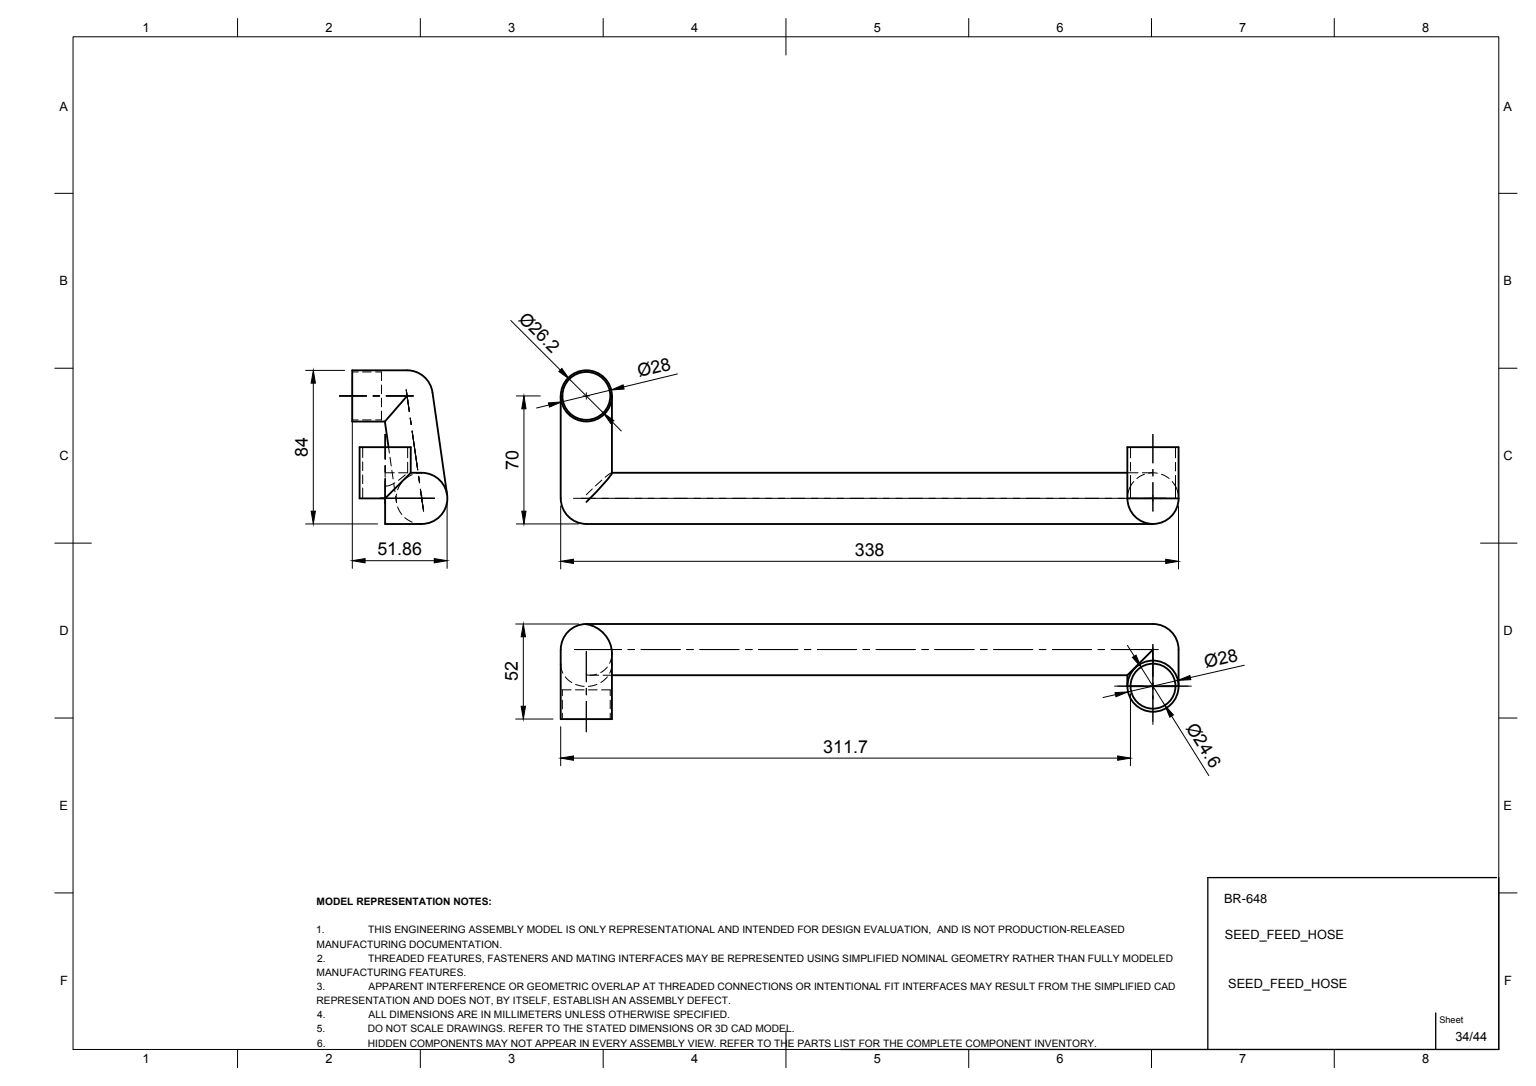
ISO-10303-21;
HEADER;
FILE_DESCRIPTION((''),'2;1');
FILE_NAME('SEED_FEED_HOSE.step','2026-10-01T22:05:39-07:00',(''),(''),'','','');
FILE_SCHEMA (('AUTOMOTIVE_DESIGN { 1 0 10303 214 3 1 1 }'));
ENDSEC;
DATA;
#10=MECHANICAL_DESIGN_GEOMETRIC_PRESENTATION_REPRESENTATION('',(#632),#24628);
#353=ELLIPSE('',#15108,1.97989898732233,1.4) ;
#354=ELLIPSE('',#15114,1.97989898732233,1.4) ;
#355=ELLIPSE('',#15116,1.97989898732233,1.4) ;
#356=ELLIPSE('',#15134,1.97989898732233,1.4) ;
#357=ELLIPSE('',#15135,1.97989898732233,1.4) ;
#358=ELLIPSE('',#15137,1.85319037744393,1.4) ;
#482=SPHERICAL_SURFACE('',#15121,1.4) ;
#483=SPHERICAL_SURFACE('',#15123,1.4) ;
#484=SPHERICAL_SURFACE('',#15129,1.4) ;
#548=SHAPE_REPRESENTATION_RELATIONSHIP('SRR','None',#24821,#590) ;
#590=ADVANCED_BREP_SHAPE_REPRESENTATION('',(#671),#24611) ;
#632=STYLED_ITEM('',(#25033),#671) ;
#671=MANIFOLD_SOLID_BREP('SEED_FEED_HOSE',#13174) ;
#902=FACE_BOUND('',#4577,.T.) ;
#903=FACE_BOUND('',#4590,.T.) ;
#984=B_SPLINE_CURVE_WITH_KNOTS('',3,(#23620,#23621,#23622,#23623,#23624,
#23625,#23626,#23627,#23628,#23629,#23630,#23631,#23632,#23633,#23634,#23635,
#23636,#23637,#23638,#23639,#23640,#23641,#23642,#23643,#23644,#23645,#23646,
#23647,#23648,#23649),.UNSPECIFIED.,.F.,.F.,(4,2,2,2,2,2,2,2,2,2,2,2,2,
2,4),(-4.08940558183937,-3.82598745493601,-3.56256932803264,-3.29915120112928,
-3.03573307422591,-2.5402179325728,-2.29246036174624,-2.04470279091969,
-1.79694522009313,-1.54918764926658,-1.05367250761347,-0.7902543807101,
-0.526836253806733,-0.263418126903367,0.),.UNSPECIFIED.) ;
#1668=LINE('',#23601,#2504) ;
#1669=LINE('',#23605,#2505) ;
#1670=LINE('',#23610,#2506) ;
#1671=LINE('',#23614,#2507) ;
#1672=LINE('',#23616,#2508) ;
#1673=LINE('',#23618,#2509) ;
#1674=LINE('',#23654,#2510) ;
#1675=LINE('',#23686,#2511) ;
#1676=LINE('',#23690,#2512) ;
#1677=LINE('',#23694,#2513) ;
#1678=LINE('',#23699,#2514) ;
#2504=VECTOR('',#18961,1.) ;
#2505=VECTOR('',#18964,1.) ;
#2506=VECTOR('',#18971,1.4) ;
#2507=VECTOR('',#18976,1.) ;
#2508=VECTOR('',#18977,1.) ;
#2509=VECTOR('',#18978,1.23) ;
#2510=VECTOR('',#18987,1.4) ;
#2511=VECTOR('',#19028,1.4) ;
#2512=VECTOR('',#19035,1.4) ;
#2513=VECTOR('',#19040,1.31) ;
#2514=VECTOR('',#19047,1.4) ;
#2905=CYLINDRICAL_SURFACE('',#15106,1.4) ;
#2906=CYLINDRICAL_SURFACE('',#15109,1.23) ;
#2907=CYLINDRICAL_SURFACE('',#15112,1.4) ;
#2908=CYLINDRICAL_SURFACE('',#15117,1.4) ;
#2909=CYLINDRICAL_SURFACE('',#15133,1.4) ;
#2910=CYLINDRICAL_SURFACE('',#15136,1.4) ;
#2911=CYLINDRICAL_SURFACE('',#15138,1.31) ;
#2912=CYLINDRICAL_SURFACE('',#15140,1.4) ;
#3590=FACE_OUTER_BOUND('',#4573,.T.) ;
#3591=FACE_OUTER_BOUND('',#4574,.T.) ;
#3592=FACE_OUTER_BOUND('',#4575,.T.) ;
#3593=FACE_OUTER_BOUND('',#4576,.T.) ;
#3594=FACE_OUTER_BOUND('',#4578,.T.) ;
#3595=FACE_OUTER_BOUND('',#4579,.T.) ;
#3596=FACE_OUTER_BOUND('',#4580,.T.) ;
#3597=FACE_OUTER_BOUND('',#4581,.T.) ;
#3598=FACE_OUTER_BOUND('',#4582,.T.) ;
#3599=FACE_OUTER_BOUND('',#4583,.T.) ;
#3600=FACE_OUTER_BOUND('',#4584,.T.) ;
#3601=FACE_OUTER_BOUND('',#4585,.T.) ;
#3602=FACE_OUTER_BOUND('',#4586,.T.) ;
#3603=FACE_OUTER_BOUND('',#4587,.T.) ;
#3604=FACE_OUTER_BOUND('',#4588,.T.) ;
#3605=FACE_OUTER_BOUND('',#4589,.T.) ;
#4573=EDGE_LOOP('',(#11423,#11424,#11425,#11426)) ;
#4574=EDGE_LOOP('',(#11427,#11428,#11429,#11430,#11431)) ;
#4575=EDGE_LOOP('',(#11432,#11433,#11434,#11435,#11436,#11437,#11438)) ;
#4576=EDGE_LOOP('',(#11439)) ;
#4577=EDGE_LOOP('',(#11440)) ;
#4578=EDGE_LOOP('',(#11441,#11442,#11443,#11444,#11445,#11446,#11447)) ;
#4579=EDGE_LOOP('',(#11448,#11449)) ;
#4580=EDGE_LOOP('',(#11450)) ;
#4581=EDGE_LOOP('',(#11451,#11452)) ;
#4582=EDGE_LOOP('',(#11453,#11454,#11455,#11456,#11457,#11458)) ;
#4583=EDGE_LOOP('',(#11459,#11460)) ;
#4584=EDGE_LOOP('',(#11461,#11462,#11463,#11464,#11465,#11466)) ;
#4585=EDGE_LOOP('',(#11467,#11468,#11469,#11470,#11471,#11472,#11473,#11474,
#11475)) ;
#4586=EDGE_LOOP('',(#11476,#11477,#11478,#11479,#11480,#11481,#11482,#11483)) ;
#4587=EDGE_LOOP('',(#11484,#11485,#11486,#11487)) ;
#4588=EDGE_LOOP('',(#11488,#11489,#11490,#11491,#11492)) ;
#4589=EDGE_LOOP('',(#11493)) ;
#4590=EDGE_LOOP('',(#11494)) ;
#5443=CIRCLE('',#15104,1.4) ;
#5444=CIRCLE('',#15105,1.23) ;
#5445=CIRCLE('',#15107,1.4) ;
#5446=CIRCLE('',#15110,1.23) ;
#5447=CIRCLE('',#15113,1.4) ;
#5448=CIRCLE('',#15115,1.4) ;
#5449=CIRCLE('',#15118,1.4) ;
#5450=CIRCLE('',#15120,1.31) ;
#5451=CIRCLE('',#15122,1.4) ;
#5452=CIRCLE('',#15124,1.4) ;
#5453=CIRCLE('',#15125,1.4) ;
#5454=CIRCLE('',#15126,1.4) ;
#5455=CIRCLE('',#15127,1.4) ;
#5456=CIRCLE('',#15128,1.4) ;
#5457=CIRCLE('',#15130,1.4) ;
#5458=CIRCLE('',#15131,1.4) ;
#5459=CIRCLE('',#15139,1.31) ;
#5460=CIRCLE('',#15141,1.4) ;
#6545=VERTEX_POINT('',#23599) ;
#6546=VERTEX_POINT('',#23600) ;
#6547=VERTEX_POINT('',#23602) ;
#6548=VERTEX_POINT('',#23604) ;
#6549=VERTEX_POINT('',#23608) ;
#6550=VERTEX_POINT('',#23613) ;
#6551=VERTEX_POINT('',#23615) ;
#6552=VERTEX_POINT('',#23617) ;
#6553=VERTEX_POINT('',#23653) ;
#6554=VERTEX_POINT('',#23655) ;
#6555=VERTEX_POINT('',#23657) ;
#6556=VERTEX_POINT('',#23663) ;
#6557=VERTEX_POINT('',#23668) ;
#6558=VERTEX_POINT('',#23669) ;
#6559=VERTEX_POINT('',#23671) ;
#6560=VERTEX_POINT('',#23673) ;
#6561=VERTEX_POINT('',#23675) ;
#6562=VERTEX_POINT('',#23679) ;
#6563=VERTEX_POINT('',#23680) ;
#6564=VERTEX_POINT('',#23685) ;
#6565=VERTEX_POINT('',#23693) ;
#6566=VERTEX_POINT('',#23697) ;
#8201=EDGE_CURVE('',#6545,#6546,#1668,.T.) ;
#8202=EDGE_CURVE('',#6545,#6547,#5443,.T.) ;
#8203=EDGE_CURVE('',#6548,#6547,#1669,.T.) ;
#8204=EDGE_CURVE('',#6548,#6546,#5444,.T.) ;
#8205=EDGE_CURVE('',#6549,#6549,#5445,.T.) ;
#8206=EDGE_CURVE('',#6549,#6547,#1670,.T.) ;
#8207=EDGE_CURVE('',#6547,#6545,#353,.T.) ;
#8208=EDGE_CURVE('',#6546,#6550,#1671,.T.) ;
#8209=EDGE_CURVE('',#6551,#6548,#1672,.T.) ;
#8210=EDGE_CURVE('',#6551,#6552,#1673,.T.) ;
#8211=EDGE_CURVE('',#6552,#6552,#5446,.T.) ;
#8212=EDGE_CURVE('',#6550,#6551,#984,.T.) ;
#8213=EDGE_CURVE('',#6547,#6545,#5447,.T.) ;
#8214=EDGE_CURVE('',#6547,#6553,#1674,.T.) ;
#8215=EDGE_CURVE('',#6554,#6553,#354,.T.) ;
#8216=EDGE_CURVE('',#6555,#6554,#5448,.T.) ;
#8217=EDGE_CURVE('',#6553,#6555,#355,.T.) ;
#8218=EDGE_CURVE('',#6550,#6551,#5449,.T.) ;
#8219=EDGE_CURVE('',#6556,#6556,#5450,.T.) ;
#8220=EDGE_CURVE('',#6554,#6555,#5451,.T.) ;
#8221=EDGE_CURVE('',#6557,#6558,#5452,.T.) ;
#8222=EDGE_CURVE('',#6558,#6559,#5453,.T.) ;
#8223=EDGE_CURVE('',#6558,#6560,#5454,.T.) ;
#8224=EDGE_CURVE('',#6560,#6561,#5455,.T.) ;
#8225=EDGE_CURVE('',#6561,#6557,#5456,.T.) ;
#8226=EDGE_CURVE('',#6562,#6563,#5457,.T.) ;
#8227=EDGE_CURVE('',#6563,#6562,#5458,.T.) ;
#8228=EDGE_CURVE('',#6553,#6564,#1675,.T.) ;
#8229=EDGE_CURVE('',#6560,#6564,#356,.T.) ;
#8230=EDGE_CURVE('',#6564,#6557,#357,.T.) ;
#8231=EDGE_CURVE('',#6561,#6563,#1676,.T.) ;
#8232=EDGE_CURVE('',#6563,#6562,#358,.T.) ;
#8233=EDGE_CURVE('',#6556,#6565,#1677,.T.) ;
#8234=EDGE_CURVE('',#6565,#6565,#5459,.T.) ;
#8235=EDGE_CURVE('',#6566,#6566,#5460,.T.) ;
#8236=EDGE_CURVE('',#6566,#6563,#1678,.T.) ;
#11423=ORIENTED_EDGE('',*,*,#8201,.F.) ;
#11424=ORIENTED_EDGE('',*,*,#8202,.T.) ;
#11425=ORIENTED_EDGE('',*,*,#8203,.F.) ;
#11426=ORIENTED_EDGE('',*,*,#8204,.T.) ;
#11427=ORIENTED_EDGE('',*,*,#8205,.F.) ;
#11428=ORIENTED_EDGE('',*,*,#8206,.T.) ;
#11429=ORIENTED_EDGE('',*,*,#8202,.F.) ;
#11430=ORIENTED_EDGE('',*,*,#8207,.F.) ;
#11431=ORIENTED_EDGE('',*,*,#8206,.F.) ;
#11432=ORIENTED_EDGE('',*,*,#8208,.F.) ;
#11433=ORIENTED_EDGE('',*,*,#8204,.F.) ;
#11434=ORIENTED_EDGE('',*,*,#8209,.F.) ;
#11435=ORIENTED_EDGE('',*,*,#8210,.T.) ;
#11436=ORIENTED_EDGE('',*,*,#8211,.F.) ;
#11437=ORIENTED_EDGE('',*,*,#8210,.F.) ;
#11438=ORIENTED_EDGE('',*,*,#8212,.F.) ;
#11439=ORIENTED_EDGE('',*,*,#8205,.T.) ;
#11440=ORIENTED_EDGE('',*,*,#8211,.T.) ;
#11441=ORIENTED_EDGE('',*,*,#8207,.T.) ;
#11442=ORIENTED_EDGE('',*,*,#8213,.F.) ;
#11443=ORIENTED_EDGE('',*,*,#8214,.T.) ;
#11444=ORIENTED_EDGE('',*,*,#8215,.F.) ;
#11445=ORIENTED_EDGE('',*,*,#8216,.F.) ;
#11446=ORIENTED_EDGE('',*,*,#8217,.F.) ;
#11447=ORIENTED_EDGE('',*,*,#8214,.F.) ;
#11448=ORIENTED_EDGE('',*,*,#8212,.T.) ;
#11449=ORIENTED_EDGE('',*,*,#8218,.F.) ;
#11450=ORIENTED_EDGE('',*,*,#8219,.T.) ;
#11451=ORIENTED_EDGE('',*,*,#8216,.T.) ;
#11452=ORIENTED_EDGE('',*,*,#8220,.T.) ;
#11453=ORIENTED_EDGE('',*,*,#8221,.T.) ;
#11454=ORIENTED_EDGE('',*,*,#8222,.T.) ;
#11455=ORIENTED_EDGE('',*,*,#8222,.F.) ;
#11456=ORIENTED_EDGE('',*,*,#8223,.T.) ;
#11457=ORIENTED_EDGE('',*,*,#8224,.T.) ;
#11458=ORIENTED_EDGE('',*,*,#8225,.T.) ;
#11459=ORIENTED_EDGE('',*,*,#8226,.T.) ;
#11460=ORIENTED_EDGE('',*,*,#8227,.T.) ;
#11461=ORIENTED_EDGE('',*,*,#8208,.T.) ;
#11462=ORIENTED_EDGE('',*,*,#8218,.T.) ;
#11463=ORIENTED_EDGE('',*,*,#8209,.T.) ;
#11464=ORIENTED_EDGE('',*,*,#8203,.T.) ;
#11465=ORIENTED_EDGE('',*,*,#8213,.T.) ;
#11466=ORIENTED_EDGE('',*,*,#8201,.T.) ;
#11467=ORIENTED_EDGE('',*,*,#8215,.T.) ;
#11468=ORIENTED_EDGE('',*,*,#8228,.T.) ;
#11469=ORIENTED_EDGE('',*,*,#8229,.F.) ;
#11470=ORIENTED_EDGE('',*,*,#8223,.F.) ;
#11471=ORIENTED_EDGE('',*,*,#8221,.F.) ;
#11472=ORIENTED_EDGE('',*,*,#8230,.F.) ;
#11473=ORIENTED_EDGE('',*,*,#8228,.F.) ;
#11474=ORIENTED_EDGE('',*,*,#8217,.T.) ;
#11475=ORIENTED_EDGE('',*,*,#8220,.F.) ;
#11476=ORIENTED_EDGE('',*,*,#8229,.T.) ;
#11477=ORIENTED_EDGE('',*,*,#8230,.T.) ;
#11478=ORIENTED_EDGE('',*,*,#8225,.F.) ;
#11479=ORIENTED_EDGE('',*,*,#8231,.T.) ;
#11480=ORIENTED_EDGE('',*,*,#8226,.F.) ;
#11481=ORIENTED_EDGE('',*,*,#8232,.F.) ;
#11482=ORIENTED_EDGE('',*,*,#8231,.F.) ;
#11483=ORIENTED_EDGE('',*,*,#8224,.F.) ;
#11484=ORIENTED_EDGE('',*,*,#8219,.F.) ;
#11485=ORIENTED_EDGE('',*,*,#8233,.T.) ;
#11486=ORIENTED_EDGE('',*,*,#8234,.F.) ;
#11487=ORIENTED_EDGE('',*,*,#8233,.F.) ;
#11488=ORIENTED_EDGE('',*,*,#8235,.F.) ;
#11489=ORIENTED_EDGE('',*,*,#8236,.T.) ;
#11490=ORIENTED_EDGE('',*,*,#8232,.T.) ;
#11491=ORIENTED_EDGE('',*,*,#8227,.F.) ;
#11492=ORIENTED_EDGE('',*,*,#8236,.F.) ;
#11493=ORIENTED_EDGE('',*,*,#8235,.T.) ;
#11494=ORIENTED_EDGE('',*,*,#8234,.T.) ;
#12270=PLANE('',#15103) ;
#12271=PLANE('',#15111) ;
#12272=PLANE('',#15119) ;
#12273=PLANE('',#15132) ;
#12274=PLANE('',#15142) ;
#12985=ADVANCED_FACE('',(#3590),#12270,.T.) ;
#12986=ADVANCED_FACE('',(#3591),#2905,.T.) ;
#12987=ADVANCED_FACE('',(#3592),#2906,.F.) ;
#12988=ADVANCED_FACE('',(#3593,#902),#12271,.T.) ;
#12989=ADVANCED_FACE('',(#3594),#2907,.T.) ;
#12990=ADVANCED_FACE('',(#3595),#2908,.T.) ;
#12991=ADVANCED_FACE('',(#3596),#12272,.T.) ;
#12992=ADVANCED_FACE('',(#3597),#482,.T.) ;
#12993=ADVANCED_FACE('',(#3598),#483,.T.) ;
#12994=ADVANCED_FACE('',(#3599),#484,.T.) ;
#12995=ADVANCED_FACE('',(#3600),#12273,.T.) ;
#12996=ADVANCED_FACE('',(#3601),#2909,.T.) ;
#12997=ADVANCED_FACE('',(#3602),#2910,.T.) ;
#12998=ADVANCED_FACE('',(#3603),#2911,.F.) ;
#12999=ADVANCED_FACE('',(#3604),#2912,.T.) ;
#13000=ADVANCED_FACE('',(#3605,#903),#12274,.T.) ;
#13174=CLOSED_SHELL('',(#12985,#12986,#12987,#12988,#12989,#12990,#12991,
#12992,#12993,#12994,#12995,#12996,#12997,#12998,#12999,#13000)) ;
#15102=AXIS2_PLACEMENT_3D('',#23597,#18957,#18958) ;
#15103=AXIS2_PLACEMENT_3D('',#23598,#18959,#18960) ;
#15104=AXIS2_PLACEMENT_3D('',#23603,#18962,#18963) ;
#15105=AXIS2_PLACEMENT_3D('',#23606,#18965,#18966) ;
#15106=AXIS2_PLACEMENT_3D('',#23607,#18967,#18968) ;
#15107=AXIS2_PLACEMENT_3D('',#23609,#18969,#18970) ;
#15108=AXIS2_PLACEMENT_3D('',#23611,#18972,#18973) ;
#15109=AXIS2_PLACEMENT_3D('',#23612,#18974,#18975) ;
#15110=AXIS2_PLACEMENT_3D('',#23619,#18979,#18980) ;
#15111=AXIS2_PLACEMENT_3D('',#23650,#18981,#18982) ;
#15112=AXIS2_PLACEMENT_3D('',#23651,#18983,#18984) ;
#15113=AXIS2_PLACEMENT_3D('',#23652,#18985,#18986) ;
#15114=AXIS2_PLACEMENT_3D('',#23656,#18988,#18989) ;
#15115=AXIS2_PLACEMENT_3D('',#23658,#18990,#18991) ;
#15116=AXIS2_PLACEMENT_3D('',#23659,#18992,#18993) ;
#15117=AXIS2_PLACEMENT_3D('',#23660,#18994,#18995) ;
#15118=AXIS2_PLACEMENT_3D('',#23661,#18996,#18997) ;
#15119=AXIS2_PLACEMENT_3D('',#23662,#18998,#18999) ;
#15120=AXIS2_PLACEMENT_3D('',#23664,#19000,#19001) ;
#15121=AXIS2_PLACEMENT_3D('',#23665,#19002,#19003) ;
#15122=AXIS2_PLACEMENT_3D('',#23666,#19004,#19005) ;
#15123=AXIS2_PLACEMENT_3D('',#23667,#19006,#19007) ;
#15124=AXIS2_PLACEMENT_3D('',#23670,#19008,#19009) ;
#15125=AXIS2_PLACEMENT_3D('',#23672,#19010,#19011) ;
#15126=AXIS2_PLACEMENT_3D('',#23674,#19012,#19013) ;
#15127=AXIS2_PLACEMENT_3D('',#23676,#19014,#19015) ;
#15128=AXIS2_PLACEMENT_3D('',#23677,#19016,#19017) ;
#15129=AXIS2_PLACEMENT_3D('',#23678,#19018,#19019) ;
#15130=AXIS2_PLACEMENT_3D('',#23681,#19020,#19021) ;
#15131=AXIS2_PLACEMENT_3D('',#23682,#19022,#19023) ;
#15132=AXIS2_PLACEMENT_3D('',#23683,#19024,#19025) ;
#15133=AXIS2_PLACEMENT_3D('',#23684,#19026,#19027) ;
#15134=AXIS2_PLACEMENT_3D('',#23687,#19029,#19030) ;
#15135=AXIS2_PLACEMENT_3D('',#23688,#19031,#19032) ;
#15136=AXIS2_PLACEMENT_3D('',#23689,#19033,#19034) ;
#15137=AXIS2_PLACEMENT_3D('',#23691,#19036,#19037) ;
#15138=AXIS2_PLACEMENT_3D('',#23692,#19038,#19039) ;
#15139=AXIS2_PLACEMENT_3D('',#23695,#19041,#19042) ;
#15140=AXIS2_PLACEMENT_3D('',#23696,#19043,#19044) ;
#15141=AXIS2_PLACEMENT_3D('',#23698,#19045,#19046) ;
#15142=AXIS2_PLACEMENT_3D('',#23700,#19048,#19049) ;
#18957=DIRECTION('axis',(0.,0.,1.)) ;
#18958=DIRECTION('refdir',(1.,0.,0.)) ;
#18959=DIRECTION('center_axis',(0.,-1.,0.)) ;
#18960=DIRECTION('ref_axis',(-1.,0.,0.)) ;
#18961=DIRECTION('',(-1.,0.,0.)) ;
#18962=DIRECTION('center_axis',(0.,-1.,0.)) ;
#18963=DIRECTION('ref_axis',(1.,0.,0.)) ;
#18964=DIRECTION('',(-1.,0.,0.)) ;
#18965=DIRECTION('center_axis',(0.,1.,0.)) ;
#18966=DIRECTION('ref_axis',(1.,0.,0.)) ;
#18967=DIRECTION('center_axis',(0.,1.,0.)) ;
#18968=DIRECTION('ref_axis',(1.,0.,0.)) ;
#18969=DIRECTION('center_axis',(0.,1.,0.)) ;
#18970=DIRECTION('ref_axis',(1.,0.,0.)) ;
#18971=DIRECTION('',(0.,-1.,0.)) ;
#18972=DIRECTION('center_axis',(0.,-0.707106781186548,-0.707106781186548)) ;
#18973=DIRECTION('ref_axis',(0.,0.707106781186547,-0.707106781186547)) ;
#18974=DIRECTION('center_axis',(0.,1.,0.)) ;
#18975=DIRECTION('ref_axis',(1.,0.,0.)) ;
#18976=DIRECTION('',(0.,1.,0.)) ;
#18977=DIRECTION('',(0.,-1.,0.)) ;
#18978=DIRECTION('',(0.,1.,0.)) ;
#18979=DIRECTION('center_axis',(0.,-1.,0.)) ;
#18980=DIRECTION('ref_axis',(1.,0.,0.)) ;
#18981=DIRECTION('center_axis',(0.,1.,0.)) ;
#18982=DIRECTION('ref_axis',(1.,0.,0.)) ;
#18983=DIRECTION('center_axis',(0.,0.,1.)) ;
#18984=DIRECTION('ref_axis',(1.,0.,0.)) ;
#18985=DIRECTION('center_axis',(0.,0.,1.)) ;
#18986=DIRECTION('ref_axis',(1.,0.,0.)) ;
#18987=DIRECTION('',(0.,0.,-1.)) ;
#18988=DIRECTION('center_axis',(-0.707106781186548,0.,-0.707106781186547)) ;
#18989=DIRECTION('ref_axis',(0.707106781186547,0.,-0.707106781186548)) ;
#18990=DIRECTION('center_axis',(0.,0.,-1.)) ;
#18991=DIRECTION('ref_axis',(1.,0.,0.)) ;
#18992=DIRECTION('center_axis',(-0.707106781186548,0.,-0.707106781186547)) ;
#18993=DIRECTION('ref_axis',(0.707106781186547,0.,-0.707106781186548)) ;
#18994=DIRECTION('center_axis',(0.,0.,1.)) ;
#18995=DIRECTION('ref_axis',(1.,0.,0.)) ;
#18996=DIRECTION('center_axis',(0.,0.,1.)) ;
#18997=DIRECTION('ref_axis',(1.,0.,0.)) ;
#18998=DIRECTION('center_axis',(0.,0.,1.)) ;
#18999=DIRECTION('ref_axis',(-1.,0.,0.)) ;
#19000=DIRECTION('center_axis',(0.,0.,1.)) ;
#19001=DIRECTION('ref_axis',(1.,0.,0.)) ;
#19002=DIRECTION('center_axis',(0.577350269189627,0.577350269189626,0.577350269189625)) ;
#19003=DIRECTION('ref_axis',(0.707106781186548,0.,-0.707106781186548)) ;
#19004=DIRECTION('center_axis',(1.,0.,0.)) ;
#19005=DIRECTION('ref_axis',(0.,0.,-1.)) ;
#19006=DIRECTION('center_axis',(0.577350269189625,0.577350269189626,0.577350269189627)) ;
#19007=DIRECTION('ref_axis',(-0.707106781186548,0.,0.707106781186547)) ;
#19008=DIRECTION('center_axis',(-1.,0.,0.)) ;
#19009=DIRECTION('ref_axis',(0.,0.,-1.)) ;
#19010=DIRECTION('center_axis',(-0.408248290463863,0.816496580927726,-0.408248290463863)) ;
#19011=DIRECTION('ref_axis',(0.707106781186548,0.,-0.707106781186547)) ;
#19012=DIRECTION('center_axis',(-1.,0.,0.)) ;
#19013=DIRECTION('ref_axis',(0.,0.,-1.)) ;
#19014=DIRECTION('center_axis',(0.,-0.989949493661167,-0.141421356237309)) ;
#19015=DIRECTION('ref_axis',(1.,0.,0.)) ;
#19016=DIRECTION('center_axis',(0.,-0.989949493661167,-0.141421356237309)) ;
#19017=DIRECTION('ref_axis',(1.,0.,0.)) ;
#19018=DIRECTION('center_axis',(0.,0.,1.)) ;
#19019=DIRECTION('ref_axis',(1.,0.,0.)) ;
#19020=DIRECTION('center_axis',(0.,0.989949493661167,0.141421356237309)) ;
#19021=DIRECTION('ref_axis',(1.,0.,0.)) ;
#19022=DIRECTION('center_axis',(0.,0.,-1.)) ;
#19023=DIRECTION('ref_axis',(1.,0.,0.)) ;
#19024=DIRECTION('center_axis',(0.,0.,1.)) ;
#19025=DIRECTION('ref_axis',(1.,0.,0.)) ;
#19026=DIRECTION('center_axis',(1.,0.,0.)) ;
#19027=DIRECTION('ref_axis',(0.,0.,-1.)) ;
#19028=DIRECTION('',(-1.,0.,0.)) ;
#19029=DIRECTION('center_axis',(-0.707106781186548,0.7,0.1)) ;
#19030=DIRECTION('ref_axis',(-0.707106781186547,-0.7,-0.1)) ;
#19031=DIRECTION('center_axis',(-0.707106781186548,0.7,0.1)) ;
#19032=DIRECTION('ref_axis',(-0.707106781186547,-0.7,-0.1)) ;
#19033=DIRECTION('center_axis',(0.,-0.989949493661167,-0.141421356237309)) ;
#19034=DIRECTION('ref_axis',(1.,0.,0.)) ;
#19035=DIRECTION('',(0.,0.989949493661167,0.141421356237309)) ;
#19036=DIRECTION('center_axis',(0.,0.655201741360129,0.755453954995706)) ;
#19037=DIRECTION('ref_axis',(0.,-0.755453954995706,0.655201741360129)) ;
#19038=DIRECTION('center_axis',(0.,0.,1.)) ;
#19039=DIRECTION('ref_axis',(1.,0.,0.)) ;
#19040=DIRECTION('',(0.,0.,1.)) ;
#19041=DIRECTION('center_axis',(0.,0.,-1.)) ;
#19042=DIRECTION('ref_axis',(1.,0.,0.)) ;
#19043=DIRECTION('center_axis',(0.,0.,1.)) ;
#19044=DIRECTION('ref_axis',(1.,0.,0.)) ;
#19045=DIRECTION('center_axis',(0.,0.,1.)) ;
#19046=DIRECTION('ref_axis',(1.,0.,0.)) ;
#19047=DIRECTION('',(0.,0.,-1.)) ;
#19048=DIRECTION('center_axis',(0.,0.,1.)) ;
#19049=DIRECTION('ref_axis',(1.,0.,0.)) ;
#23597=CARTESIAN_POINT('',(0.,0.,0.)) ;
#23598=CARTESIAN_POINT('Origin',(8.,-7.4,-8.)) ;
#23599=CARTESIAN_POINT('',(9.4,-7.4,-8.)) ;
#23600=CARTESIAN_POINT('',(9.23,-7.4,-8.)) ;
#23601=CARTESIAN_POINT('',(8.,-7.4,-8.)) ;
#23602=CARTESIAN_POINT('',(6.6,-7.4,-8.)) ;
#23603=CARTESIAN_POINT('Origin',(8.,-7.4,-8.)) ;
#23604=CARTESIAN_POINT('',(6.77,-7.4,-8.)) ;
#23605=CARTESIAN_POINT('',(8.,-7.4,-8.)) ;
#23606=CARTESIAN_POINT('Origin',(8.,-7.4,-8.)) ;
#23607=CARTESIAN_POINT('Origin',(8.,-6.,-8.)) ;
#23608=CARTESIAN_POINT('',(6.6,-4.6,-8.)) ;
#23609=CARTESIAN_POINT('Origin',(8.,-4.6,-8.)) ;
#23610=CARTESIAN_POINT('',(6.6,-6.,-8.)) ;
#23611=CARTESIAN_POINT('Origin',(8.,-7.4,-8.)) ;
#23612=CARTESIAN_POINT('Origin',(8.,-6.,-8.)) ;
#23613=CARTESIAN_POINT('',(9.23,-6.73134463286384,-8.)) ;
#23614=CARTESIAN_POINT('',(9.23,-6.,-8.)) ;
#23615=CARTESIAN_POINT('',(6.77,-6.73134463286384,-8.)) ;
#23616=CARTESIAN_POINT('',(6.77,-6.,-8.)) ;
#23617=CARTESIAN_POINT('',(6.77,-4.6,-8.)) ;
#23618=CARTESIAN_POINT('',(6.77,-6.,-8.)) ;
#23619=CARTESIAN_POINT('Origin',(8.,-4.6,-8.)) ;
#23620=CARTESIAN_POINT('Ctrl Pts',(9.23,-6.73134463286384,-8.)) ;
#23621=CARTESIAN_POINT('Ctrl Pts',(9.23,-6.73134463286384,-8.08780604230112)) ;
#23622=CARTESIAN_POINT('Ctrl Pts',(9.22072799863506,-6.71377567825997,-8.17157966039377)) ;
#23623=CARTESIAN_POINT('Ctrl Pts',(9.18717385924031,-6.65723564339427,-8.33201605328968)) ;
#23624=CARTESIAN_POINT('Ctrl Pts',(9.16282342807417,-6.61855579361812,-8.40876702722022)) ;
#23625=CARTESIAN_POINT('Ctrl Pts',(9.10036397056989,-6.53281362355673,-8.55538171579166)) ;
#23626=CARTESIAN_POINT('Ctrl Pts',(9.06220933130718,-6.48575698731823,-8.62513175063278)) ;
#23627=CARTESIAN_POINT('Ctrl Pts',(8.97399636293542,-6.39229962882938,-8.75525456150379)) ;
#23628=CARTESIAN_POINT('Ctrl Pts',(8.92390015166212,-6.3458722876066,-8.81558253005679)) ;
#23629=CARTESIAN_POINT('Ctrl Pts',(8.76786334513407,-6.22216790150124,-8.97161933658483)) ;
#23630=CARTESIAN_POINT('Ctrl Pts',(8.63606117977349,-6.14254167736889,-9.06545127512159)) ;
#23631=CARTESIAN_POINT('Ctrl Pts',(8.41018345337793,-6.05903266002601,-9.16248210994164)) ;
#23632=CARTESIAN_POINT('Ctrl Pts',(8.33024026117397,-6.03696421286031,-9.18778520433019)) ;
#23633=CARTESIAN_POINT('Ctrl Pts',(8.16644432291491,-6.00744067465883,-9.22155172186516)) ;
#23634=CARTESIAN_POINT('Ctrl Pts',(8.08258585694218,-6.,-9.23)) ;
#23635=CARTESIAN_POINT('Ctrl Pts',(7.91741414305782,-6.,-9.23)) ;
#23636=CARTESIAN_POINT('Ctrl Pts',(7.83355567708509,-6.00744067465883,-9.22155172186516)) ;
#23637=CARTESIAN_POINT('Ctrl Pts',(7.66975973882603,-6.0369642128603,-9.18778520433019)) ;
#23638=CARTESIAN_POINT('Ctrl Pts',(7.58981654662208,-6.05903266002601,-9.16248210994164)) ;
#23639=CARTESIAN_POINT('Ctrl Pts',(7.36393882022652,-6.14254167736889,-9.06545127512159)) ;
#23640=CARTESIAN_POINT('Ctrl Pts',(7.23213665486593,-6.22216790150124,-8.97161933658483)) ;
#23641=CARTESIAN_POINT('Ctrl Pts',(7.07609984833788,-6.3458722876066,-8.81558253005679)) ;
#23642=CARTESIAN_POINT('Ctrl Pts',(7.02600363706458,-6.39229962882937,-8.75525456150379)) ;
#23643=CARTESIAN_POINT('Ctrl Pts',(6.93779066869282,-6.48575698731822,-8.62513175063279)) ;
#23644=CARTESIAN_POINT('Ctrl Pts',(6.89963602943012,-6.53281362355673,-8.55538171579166)) ;
#23645=CARTESIAN_POINT('Ctrl Pts',(6.83717657192583,-6.61855579361812,-8.40876702722023)) ;
#23646=CARTESIAN_POINT('Ctrl Pts',(6.81282614075969,-6.65723564339427,-8.33201605328968)) ;
#23647=CARTESIAN_POINT('Ctrl Pts',(6.77927200136494,-6.71377567825997,-8.17157966039377)) ;
#23648=CARTESIAN_POINT('Ctrl Pts',(6.77,-6.73134463286384,-8.08780604230112)) ;
#23649=CARTESIAN_POINT('Ctrl Pts',(6.77,-6.73134463286384,-8.)) ;
#23650=CARTESIAN_POINT('Origin',(8.,-4.6,-8.)) ;
#23651=CARTESIAN_POINT('Origin',(8.,-7.4,-9.)) ;
#23652=CARTESIAN_POINT('Origin',(8.,-7.4,-8.)) ;
#23653=CARTESIAN_POINT('',(6.6,-7.4,-8.6)) ;
#23654=CARTESIAN_POINT('',(6.6,-7.4,-9.)) ;
#23655=CARTESIAN_POINT('',(8.,-8.8,-10.)) ;
#23656=CARTESIAN_POINT('Origin',(8.,-7.4,-10.)) ;
#23657=CARTESIAN_POINT('',(8.,-6.,-10.)) ;
#23658=CARTESIAN_POINT('Origin',(8.,-7.4,-10.)) ;
#23659=CARTESIAN_POINT('Origin',(8.,-7.4,-10.)) ;
#23660=CARTESIAN_POINT('Origin',(8.,-7.4,-9.)) ;
#23661=CARTESIAN_POINT('Origin',(8.,-7.4,-8.)) ;
#23662=CARTESIAN_POINT('Origin',(-23.,-1.8,-7.8)) ;
#23663=CARTESIAN_POINT('',(-24.31,-1.8,-7.8)) ;
#23664=CARTESIAN_POINT('Origin',(-23.,-1.8,-7.8)) ;
#23665=CARTESIAN_POINT('Origin',(8.,-7.4,-10.)) ;
#23666=CARTESIAN_POINT('Origin',(8.,-7.4,-10.)) ;
#23667=CARTESIAN_POINT('Origin',(-23.,-7.4,-10.)) ;
#23668=CARTESIAN_POINT('',(-23.,-7.20201010126786,-11.3859292911256)) ;
#23669=CARTESIAN_POINT('',(-23.,-8.02609903369994,-11.2521980673999)) ;
#23670=CARTESIAN_POINT('Origin',(-23.,-7.4,-10.)) ;
#23671=CARTESIAN_POINT('',(-23.8082903768655,-8.20829037686548,-10.8082903768655)) ;
#23672=CARTESIAN_POINT('Origin',(-23.,-7.4,-10.)) ;
#23673=CARTESIAN_POINT('',(-23.,-7.59798989873238,-8.61407070887439)) ;
#23674=CARTESIAN_POINT('Origin',(-23.,-7.4,-10.)) ;
#23675=CARTESIAN_POINT('',(-24.4,-7.40000000000007,-10.)) ;
#23676=CARTESIAN_POINT('Origin',(-23.,-7.4,-10.)) ;
#23677=CARTESIAN_POINT('Origin',(-23.,-7.4,-10.)) ;
#23678=CARTESIAN_POINT('Origin',(-23.,-1.8,-9.2)) ;
#23679=CARTESIAN_POINT('',(-21.6,-1.8,-9.2)) ;
#23680=CARTESIAN_POINT('',(-24.4,-1.8,-9.2)) ;
#23681=CARTESIAN_POINT('Origin',(-23.,-1.8,-9.2)) ;
#23682=CARTESIAN_POINT('Origin',(-23.,-1.8,-9.2)) ;
#23683=CARTESIAN_POINT('Origin',(8.,-7.4,-8.)) ;
#23684=CARTESIAN_POINT('Origin',(-7.5,-7.4,-10.)) ;
#23685=CARTESIAN_POINT('',(-22.8020101012678,-7.4,-8.6)) ;
#23686=CARTESIAN_POINT('',(-7.5,-7.4,-8.6)) ;
#23687=CARTESIAN_POINT('Origin',(-23.,-7.4,-10.)) ;
#23688=CARTESIAN_POINT('Origin',(-23.,-7.4,-10.)) ;
#23689=CARTESIAN_POINT('Origin',(-23.,-4.6,-9.6)) ;
#23690=CARTESIAN_POINT('',(-24.4,-4.6,-9.6)) ;
#23691=CARTESIAN_POINT('Origin',(-23.,-1.8,-9.2)) ;
#23692=CARTESIAN_POINT('Origin',(-23.,-1.8,-7.)) ;
#23693=CARTESIAN_POINT('',(-24.31,-1.8,-6.2)) ;
#23694=CARTESIAN_POINT('',(-24.31,-1.8,-7.)) ;
#23695=CARTESIAN_POINT('Origin',(-23.,-1.8,-6.2)) ;
#23696=CARTESIAN_POINT('Origin',(-23.,-1.8,-7.)) ;
#23697=CARTESIAN_POINT('',(-24.4,-1.8,-6.2)) ;
#23698=CARTESIAN_POINT('Origin',(-23.,-1.8,-6.2)) ;
#23699=CARTESIAN_POINT('',(-24.4,-1.8,-7.)) ;
#23700=CARTESIAN_POINT('Origin',(-23.,-1.8,-6.2)) ;
#24563=UNCERTAINTY_MEASURE_WITH_UNIT(LENGTH_MEASURE(0.001),#24629,
'DISTANCE_ACCURACY_VALUE',
'Maximum model space distance between geometric entities at asserted c
onnectivities') ;
#24580=UNCERTAINTY_MEASURE_WITH_UNIT(LENGTH_MEASURE(0.001),#24629,
'DISTANCE_ACCURACY_VALUE',
'Maximum model space distance between geometric entities at asserted c
onnectivities') ;
#24611=(
GEOMETRIC_REPRESENTATION_CONTEXT(3)
GLOBAL_UNCERTAINTY_ASSIGNED_CONTEXT((#24563))
GLOBAL_UNIT_ASSIGNED_CONTEXT((#24629,#24631,#24632))
REPRESENTATION_CONTEXT('','3D')
) ;
#24628=(
GEOMETRIC_REPRESENTATION_CONTEXT(3)
GLOBAL_UNCERTAINTY_ASSIGNED_CONTEXT((#24580))
GLOBAL_UNIT_ASSIGNED_CONTEXT((#24629,#24631,#24632))
REPRESENTATION_CONTEXT('','3D')
) ;
#24629=(
LENGTH_UNIT()
NAMED_UNIT(*)
SI_UNIT(.CENTI.,.METRE.)
) ;
#24631=(
NAMED_UNIT(*)
PLANE_ANGLE_UNIT()
SI_UNIT($,.RADIAN.)
) ;
#24632=(
NAMED_UNIT(*)
SI_UNIT($,.STERADIAN.)
SOLID_ANGLE_UNIT()
) ;
#24663=SHAPE_DEFINITION_REPRESENTATION(#24732,#24821) ;
#24732=PRODUCT_DEFINITION_SHAPE('',$,#24869) ;
#24821=SHAPE_REPRESENTATION('',(#15102),#24611) ;
#24838=PRODUCT_DEFINITION_CONTEXT('part definition',#24981,'design') ;
#24869=PRODUCT_DEFINITION('SEED_FEED_HOSE','SEED_FEED_HOSE',#24916,
#24838) ;
#24916=PRODUCT_DEFINITION_FORMATION('',$,#25013) ;
#24981=APPLICATION_CONTEXT(
'Core Data for Automotive Mechanical Design Process') ;
#24982=PRODUCT_CONTEXT('part definition',#24981,'mechanical') ;
#25013=PRODUCT('SEED_FEED_HOSE','SEED_FEED_HOSE',$,(#24982)) ;
#25033=PRESENTATION_STYLE_ASSIGNMENT((#25043)) ;
#25043=SURFACE_STYLE_USAGE(.BOTH.,#25053) ;
#25053=SURFACE_SIDE_STYLE('',(#25063)) ;
#25063=SURFACE_STYLE_FILL_AREA(#25073) ;
#25073=FILL_AREA_STYLE('Rubber - Soft',(#25083)) ;
#25083=FILL_AREA_STYLE_COLOUR('Rubber - Soft',#25093) ;
#25093=COLOUR_RGB('Rubber - Soft', 0.09019608, 0.27058824, 0.51372549) ;
ENDSEC;
END-ISO-10303-21;
